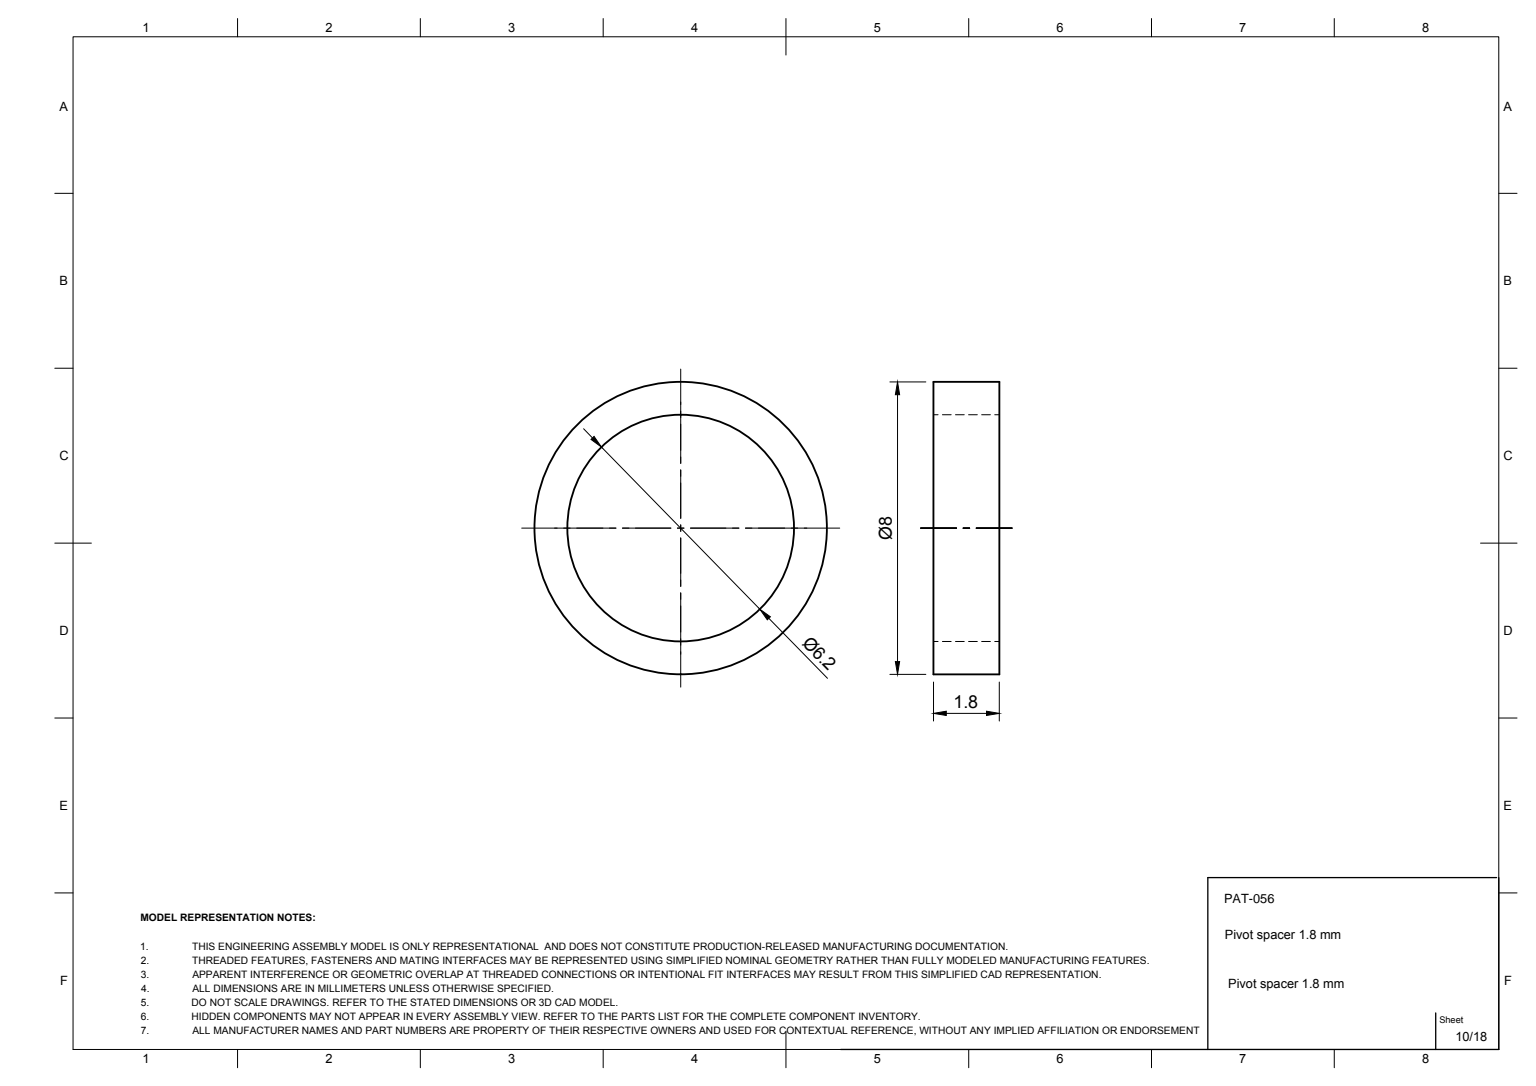
ISO-10303-21;
HEADER;
/* Generated by software containing ST-Developer
 * from STEP Tools, Inc. (www.steptools.com) 
 */

FILE_DESCRIPTION(
/* description */ ('Hook toggle clamp'),
/* implementation_level */ '2;1');

FILE_NAME(
/* name */ 'Pivot spacer 1.8 mm.step',
/* time_stamp */ '2026-10-27T21:56:56-07:00',
/* author */ (''),
/* organization */ (''),
/* preprocessor_version */ 'ST-DEVELOPER v20.2',
/* originating_system */ 'Autodesk Translation Framework v15.17.0.0',
/* authorisation */ '');

FILE_SCHEMA (('AUTOMOTIVE_DESIGN { 1 0 10303 214 3 1 1 }'));
ENDSEC;

DATA;
#10=MECHANICAL_DESIGN_GEOMETRIC_PRESENTATION_REPRESENTATION('',(#193),#5458);
#159=SHAPE_REPRESENTATION_RELATIONSHIP('SRR','None',#5541,#176);
#176=ADVANCED_BREP_SHAPE_REPRESENTATION('',(#210),#5443);
#193=STYLED_ITEM('',(#5710),#210);
#210=MANIFOLD_SOLID_BREP('Body1',#2974);
#249=FACE_BOUND('',#670,.T.);
#250=FACE_BOUND('',#672,.T.);
#334=PLANE('',#3303);
#335=PLANE('',#3304);
#467=FACE_OUTER_BOUND('',#667,.T.);
#468=FACE_OUTER_BOUND('',#668,.T.);
#469=FACE_OUTER_BOUND('',#669,.T.);
#470=FACE_OUTER_BOUND('',#671,.T.);
#667=EDGE_LOOP('',(#2365,#2366,#2367,#2368));
#668=EDGE_LOOP('',(#2369,#2370,#2371,#2372));
#669=EDGE_LOOP('',(#2373));
#670=EDGE_LOOP('',(#2374));
#671=EDGE_LOOP('',(#2375));
#672=EDGE_LOOP('',(#2376));
#932=LINE('',#4819,#1169);
#933=LINE('',#4825,#1170);
#1169=VECTOR('',#3894,0.31);
#1170=VECTOR('',#3901,0.4);
#1308=CIRCLE('',#3298,0.31);
#1309=CIRCLE('',#3299,0.31);
#1310=CIRCLE('',#3301,0.4);
#1311=CIRCLE('',#3302,0.4);
#1503=VERTEX_POINT('',#4816);
#1504=VERTEX_POINT('',#4818);
#1505=VERTEX_POINT('',#4822);
#1506=VERTEX_POINT('',#4824);
#1809=EDGE_CURVE('',#1503,#1503,#1308,.T.);
#1810=EDGE_CURVE('',#1503,#1504,#932,.T.);
#1811=EDGE_CURVE('',#1504,#1504,#1309,.T.);
#1812=EDGE_CURVE('',#1505,#1505,#1310,.T.);
#1813=EDGE_CURVE('',#1505,#1506,#933,.T.);
#1814=EDGE_CURVE('',#1506,#1506,#1311,.T.);
#2365=ORIENTED_EDGE('',*,*,#1809,.F.);
#2366=ORIENTED_EDGE('',*,*,#1810,.T.);
#2367=ORIENTED_EDGE('',*,*,#1811,.T.);
#2368=ORIENTED_EDGE('',*,*,#1810,.F.);
#2369=ORIENTED_EDGE('',*,*,#1812,.F.);
#2370=ORIENTED_EDGE('',*,*,#1813,.T.);
#2371=ORIENTED_EDGE('',*,*,#1814,.T.);
#2372=ORIENTED_EDGE('',*,*,#1813,.F.);
#2373=ORIENTED_EDGE('',*,*,#1812,.T.);
#2374=ORIENTED_EDGE('',*,*,#1809,.T.);
#2375=ORIENTED_EDGE('',*,*,#1814,.F.);
#2376=ORIENTED_EDGE('',*,*,#1811,.F.);
#2766=CYLINDRICAL_SURFACE('',#3297,0.31);
#2767=CYLINDRICAL_SURFACE('',#3300,0.4);
#2871=ADVANCED_FACE('',(#467),#2766,.F.);
#2872=ADVANCED_FACE('',(#468),#2767,.T.);
#2873=ADVANCED_FACE('',(#469,#249),#334,.T.);
#2874=ADVANCED_FACE('',(#470,#250),#335,.F.);
#2974=CLOSED_SHELL('',(#2871,#2872,#2873,#2874));
#3296=AXIS2_PLACEMENT_3D('',#4814,#3888,#3889);
#3297=AXIS2_PLACEMENT_3D('',#4815,#3890,#3891);
#3298=AXIS2_PLACEMENT_3D('',#4817,#3892,#3893);
#3299=AXIS2_PLACEMENT_3D('',#4820,#3895,#3896);
#3300=AXIS2_PLACEMENT_3D('',#4821,#3897,#3898);
#3301=AXIS2_PLACEMENT_3D('',#4823,#3899,#3900);
#3302=AXIS2_PLACEMENT_3D('',#4826,#3902,#3903);
#3303=AXIS2_PLACEMENT_3D('',#4827,#3904,#3905);
#3304=AXIS2_PLACEMENT_3D('',#4828,#3906,#3907);
#3888=DIRECTION('axis',(0.,0.,1.));
#3889=DIRECTION('refdir',(1.,0.,0.));
#3890=DIRECTION('center_axis',(0.,1.,0.));
#3891=DIRECTION('ref_axis',(1.,0.,0.));
#3892=DIRECTION('center_axis',(0.,-1.,0.));
#3893=DIRECTION('ref_axis',(1.,0.,0.));
#3894=DIRECTION('',(0.,-1.,0.));
#3895=DIRECTION('center_axis',(0.,-1.,0.));
#3896=DIRECTION('ref_axis',(1.,0.,0.));
#3897=DIRECTION('center_axis',(0.,1.,0.));
#3898=DIRECTION('ref_axis',(1.,0.,0.));
#3899=DIRECTION('center_axis',(0.,1.,0.));
#3900=DIRECTION('ref_axis',(1.,0.,0.));
#3901=DIRECTION('',(0.,-1.,0.));
#3902=DIRECTION('center_axis',(0.,1.,0.));
#3903=DIRECTION('ref_axis',(1.,0.,0.));
#3904=DIRECTION('center_axis',(0.,1.,0.));
#3905=DIRECTION('ref_axis',(1.,0.,0.));
#3906=DIRECTION('center_axis',(0.,1.,0.));
#3907=DIRECTION('ref_axis',(1.,0.,0.));
#4814=CARTESIAN_POINT('',(0.,0.,0.));
#4815=CARTESIAN_POINT('Origin',(-2.49048674522936,-0.74,2.28211064313086));
#4816=CARTESIAN_POINT('',(-2.80048674522936,-0.56,2.28211064313086));
#4817=CARTESIAN_POINT('Origin',(-2.49048674522936,-0.56,2.28211064313086));
#4818=CARTESIAN_POINT('',(-2.80048674522936,-0.74,2.28211064313086));
#4819=CARTESIAN_POINT('',(-2.80048674522936,-0.74,2.28211064313086));
#4820=CARTESIAN_POINT('Origin',(-2.49048674522936,-0.74,2.28211064313086));
#4821=CARTESIAN_POINT('Origin',(-2.49048674522936,-0.74,2.28211064313086));
#4822=CARTESIAN_POINT('',(-2.89048674522936,-0.56,2.28211064313086));
#4823=CARTESIAN_POINT('Origin',(-2.49048674522936,-0.56,2.28211064313086));
#4824=CARTESIAN_POINT('',(-2.89048674522936,-0.74,2.28211064313086));
#4825=CARTESIAN_POINT('',(-2.89048674522936,-0.74,2.28211064313086));
#4826=CARTESIAN_POINT('Origin',(-2.49048674522936,-0.74,2.28211064313086));
#4827=CARTESIAN_POINT('Origin',(-2.49048674522936,-0.56,2.28211064313086));
#4828=CARTESIAN_POINT('Origin',(-2.49048674522936,-0.74,2.28211064313086));
#5420=UNCERTAINTY_MEASURE_WITH_UNIT(LENGTH_MEASURE(0.001),#5459,
'DISTANCE_ACCURACY_VALUE',
'Maximum model space distance between geometric entities at asserted c
onnectivities');
#5435=UNCERTAINTY_MEASURE_WITH_UNIT(LENGTH_MEASURE(0.001),#5459,
'DISTANCE_ACCURACY_VALUE',
'Maximum model space distance between geometric entities at asserted c
onnectivities');
#5443=(
GEOMETRIC_REPRESENTATION_CONTEXT(3)
GLOBAL_UNCERTAINTY_ASSIGNED_CONTEXT((#5420))
GLOBAL_UNIT_ASSIGNED_CONTEXT((#5459,#5461,#5462))
REPRESENTATION_CONTEXT('','3D')
);
#5458=(
GEOMETRIC_REPRESENTATION_CONTEXT(3)
GLOBAL_UNCERTAINTY_ASSIGNED_CONTEXT((#5435))
GLOBAL_UNIT_ASSIGNED_CONTEXT((#5459,#5461,#5462))
REPRESENTATION_CONTEXT('','3D')
);
#5459=(
LENGTH_UNIT()
NAMED_UNIT(*)
SI_UNIT(.CENTI.,.METRE.)
);
#5461=(
NAMED_UNIT(*)
PLANE_ANGLE_UNIT()
SI_UNIT($,.RADIAN.)
);
#5462=(
NAMED_UNIT(*)
SI_UNIT($,.STERADIAN.)
SOLID_ANGLE_UNIT()
);
#5470=SHAPE_DEFINITION_REPRESENTATION(#5492,#5541);
#5492=PRODUCT_DEFINITION_SHAPE('',$,#5564);
#5541=SHAPE_REPRESENTATION('',(#3296),#5443);
#5556=PRODUCT_DEFINITION_CONTEXT('part definition',#5624,'design');
#5564=PRODUCT_DEFINITION('Pivot spacer 1.8 mm','Pivot spacer 1.8 mm',#5586,
#5556);
#5586=PRODUCT_DEFINITION_FORMATION('',$,#5633);
#5624=APPLICATION_CONTEXT(
'Core Data for Automotive Mechanical Design Process');
#5625=PRODUCT_CONTEXT('part definition',#5624,'mechanical');
#5633=PRODUCT('Pivot spacer 1.8 mm','Pivot spacer 1.8 mm',
'Pivot spacer 1.8 mm',(#5625));
#5704=COLOUR_RGB('Sky Blue',0.24,0.69,0.87);
#5705=FILL_AREA_STYLE_COLOUR('',#5704);
#5706=FILL_AREA_STYLE('',(#5705));
#5707=SURFACE_STYLE_FILL_AREA(#5706);
#5708=SURFACE_SIDE_STYLE('',(#5707));
#5709=SURFACE_STYLE_USAGE(.BOTH.,#5708);
#5710=PRESENTATION_STYLE_ASSIGNMENT((#5709));
ENDSEC;
END-ISO-10303-21;
